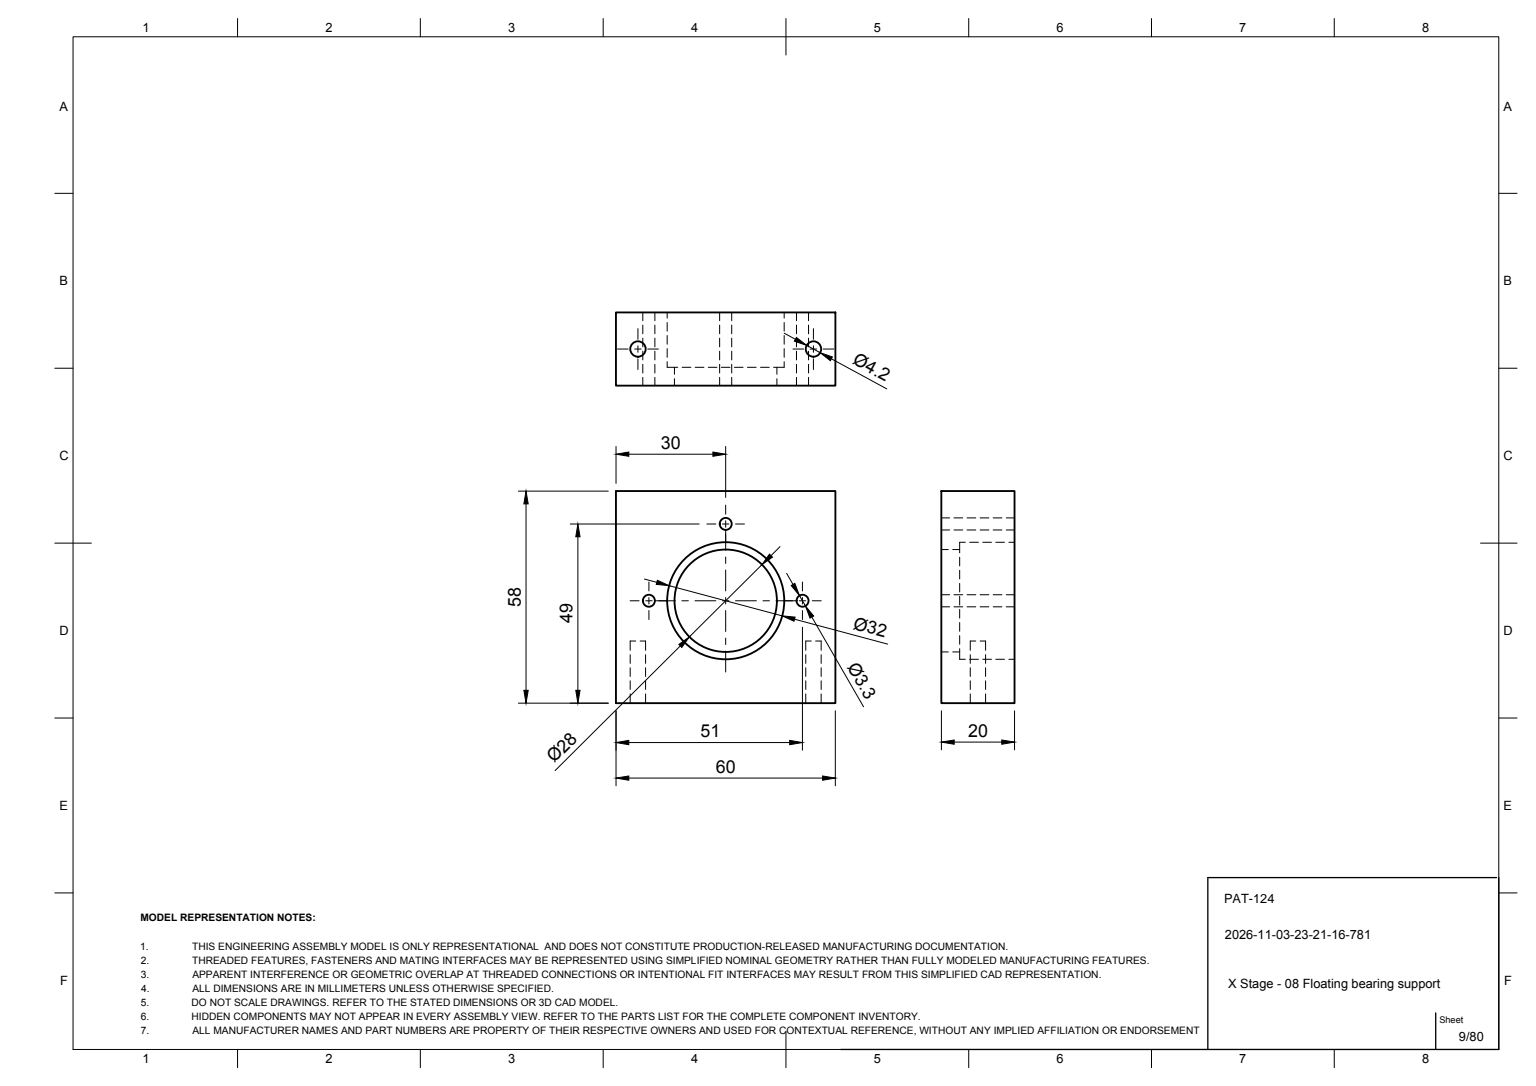
ISO-10303-21;
HEADER;
/* Generated by software containing ST-Developer
 * from STEP Tools, Inc. (www.steptools.com) 
 */

FILE_DESCRIPTION(
/* description */ ('XY cross-slide table'),
/* implementation_level */ '2;1');

FILE_NAME(
/* name */ 'X Stage - 08 Floating bearing support.step',
/* time_stamp */ '2026-10-28T03:22:46-07:00',
/* author */ (''),
/* organization */ (''),
/* preprocessor_version */ 'ST-DEVELOPER v20.2',
/* originating_system */ 'Autodesk Translation Framework v15.17.0.0',
/* authorisation */ '');

FILE_SCHEMA (('AUTOMOTIVE_DESIGN { 1 0 10303 214 3 1 1 }'));
ENDSEC;

DATA;
#10=MECHANICAL_DESIGN_GEOMETRIC_PRESENTATION_REPRESENTATION('',(#1674),#62984);
#1508=SHAPE_REPRESENTATION_RELATIONSHIP('SRR','None',#63356,#1591);
#1591=ADVANCED_BREP_SHAPE_REPRESENTATION('',(#1787),#62893);
#1674=STYLED_ITEM('',(#63912),#1787);
#1787=MANIFOLD_SOLID_BREP('Body1',#22968);
#1925=FACE_BOUND('',#4278,.T.);
#1926=FACE_BOUND('',#4286,.T.);
#1927=FACE_BOUND('',#4287,.T.);
#1928=FACE_BOUND('',#4288,.T.);
#1929=FACE_BOUND('',#4289,.T.);
#1930=FACE_BOUND('',#4292,.T.);
#1931=FACE_BOUND('',#4293,.T.);
#1932=FACE_BOUND('',#4294,.T.);
#1933=FACE_BOUND('',#4295,.T.);
#1934=FACE_BOUND('',#4298,.T.);
#1935=FACE_BOUND('',#4299,.T.);
#2324=PLANE('',#24120);
#2325=PLANE('',#24127);
#2326=PLANE('',#24131);
#2327=PLANE('',#24132);
#2328=PLANE('',#24133);
#2329=PLANE('',#24134);
#2330=PLANE('',#24135);
#2331=PLANE('',#24136);
#2332=PLANE('',#24137);
#2921=FACE_OUTER_BOUND('',#4273,.T.);
#2922=FACE_OUTER_BOUND('',#4274,.T.);
#2923=FACE_OUTER_BOUND('',#4275,.T.);
#2924=FACE_OUTER_BOUND('',#4276,.T.);
#2925=FACE_OUTER_BOUND('',#4277,.T.);
#2926=FACE_OUTER_BOUND('',#4279,.T.);
#2927=FACE_OUTER_BOUND('',#4280,.T.);
#2928=FACE_OUTER_BOUND('',#4281,.T.);
#2929=FACE_OUTER_BOUND('',#4282,.T.);
#2930=FACE_OUTER_BOUND('',#4283,.T.);
#2931=FACE_OUTER_BOUND('',#4284,.T.);
#2932=FACE_OUTER_BOUND('',#4285,.T.);
#2933=FACE_OUTER_BOUND('',#4290,.T.);
#2934=FACE_OUTER_BOUND('',#4291,.T.);
#2935=FACE_OUTER_BOUND('',#4296,.T.);
#2936=FACE_OUTER_BOUND('',#4297,.T.);
#4273=EDGE_LOOP('',(#15152,#15153,#15154,#15155));
#4274=EDGE_LOOP('',(#15156,#15157,#15158,#15159));
#4275=EDGE_LOOP('',(#15160,#15161,#15162,#15163));
#4276=EDGE_LOOP('',(#15164,#15165,#15166,#15167));
#4277=EDGE_LOOP('',(#15168));
#4278=EDGE_LOOP('',(#15169));
#4279=EDGE_LOOP('',(#15170,#15171,#15172,#15173));
#4280=EDGE_LOOP('',(#15174,#15175,#15176,#15177));
#4281=EDGE_LOOP('',(#15178));
#4282=EDGE_LOOP('',(#15179,#15180,#15181,#15182));
#4283=EDGE_LOOP('',(#15183));
#4284=EDGE_LOOP('',(#15184,#15185,#15186,#15187));
#4285=EDGE_LOOP('',(#15188,#15189,#15190,#15191));
#4286=EDGE_LOOP('',(#15192));
#4287=EDGE_LOOP('',(#15193));
#4288=EDGE_LOOP('',(#15194));
#4289=EDGE_LOOP('',(#15195));
#4290=EDGE_LOOP('',(#15196,#15197,#15198,#15199));
#4291=EDGE_LOOP('',(#15200,#15201,#15202,#15203));
#4292=EDGE_LOOP('',(#15204));
#4293=EDGE_LOOP('',(#15205));
#4294=EDGE_LOOP('',(#15206));
#4295=EDGE_LOOP('',(#15207));
#4296=EDGE_LOOP('',(#15208,#15209,#15210,#15211));
#4297=EDGE_LOOP('',(#15212,#15213,#15214,#15215));
#4298=EDGE_LOOP('',(#15216));
#4299=EDGE_LOOP('',(#15217));
#5982=LINE('',#33138,#7469);
#5983=LINE('',#33144,#7470);
#5984=LINE('',#33150,#7471);
#5985=LINE('',#33156,#7472);
#5986=LINE('',#33163,#7473);
#5987=LINE('',#33169,#7474);
#5988=LINE('',#33176,#7475);
#5989=LINE('',#33182,#7476);
#5990=LINE('',#33184,#7477);
#5991=LINE('',#33186,#7478);
#5992=LINE('',#33187,#7479);
#5993=LINE('',#33190,#7480);
#5994=LINE('',#33192,#7481);
#5995=LINE('',#33193,#7482);
#5996=LINE('',#33196,#7483);
#5997=LINE('',#33198,#7484);
#5998=LINE('',#33199,#7485);
#5999=LINE('',#33201,#7486);
#6000=LINE('',#33202,#7487);
#7469=VECTOR('',#26757,0.165);
#7470=VECTOR('',#26764,0.165);
#7471=VECTOR('',#26771,0.165);
#7472=VECTOR('',#26778,1.6);
#7473=VECTOR('',#26787,1.4);
#7474=VECTOR('',#26794,0.21);
#7475=VECTOR('',#26803,0.21);
#7476=VECTOR('',#26810,1.);
#7477=VECTOR('',#26811,1.);
#7478=VECTOR('',#26812,1.);
#7479=VECTOR('',#26813,1.);
#7480=VECTOR('',#26816,1.);
#7481=VECTOR('',#26817,1.);
#7482=VECTOR('',#26818,1.);
#7483=VECTOR('',#26821,1.);
#7484=VECTOR('',#26822,1.);
#7485=VECTOR('',#26823,1.);
#7486=VECTOR('',#26826,1.);
#7487=VECTOR('',#26827,1.);
#8928=CIRCLE('',#24109,0.165);
#8929=CIRCLE('',#24110,0.165);
#8930=CIRCLE('',#24112,0.165);
#8931=CIRCLE('',#24113,0.165);
#8932=CIRCLE('',#24115,0.165);
#8933=CIRCLE('',#24116,0.165);
#8934=CIRCLE('',#24118,1.6);
#8935=CIRCLE('',#24119,1.6);
#8936=CIRCLE('',#24121,1.4);
#8937=CIRCLE('',#24123,1.4);
#8938=CIRCLE('',#24125,0.21);
#8939=CIRCLE('',#24126,0.21);
#8940=CIRCLE('',#24129,0.21);
#8941=CIRCLE('',#24130,0.21);
#9853=VERTEX_POINT('',#33135);
#9854=VERTEX_POINT('',#33137);
#9855=VERTEX_POINT('',#33141);
#9856=VERTEX_POINT('',#33143);
#9857=VERTEX_POINT('',#33147);
#9858=VERTEX_POINT('',#33149);
#9859=VERTEX_POINT('',#33153);
#9860=VERTEX_POINT('',#33155);
#9861=VERTEX_POINT('',#33159);
#9862=VERTEX_POINT('',#33162);
#9863=VERTEX_POINT('',#33166);
#9864=VERTEX_POINT('',#33168);
#9865=VERTEX_POINT('',#33173);
#9866=VERTEX_POINT('',#33175);
#9867=VERTEX_POINT('',#33180);
#9868=VERTEX_POINT('',#33181);
#9869=VERTEX_POINT('',#33183);
#9870=VERTEX_POINT('',#33185);
#9871=VERTEX_POINT('',#33189);
#9872=VERTEX_POINT('',#33191);
#9873=VERTEX_POINT('',#33195);
#9874=VERTEX_POINT('',#33197);
#11960=EDGE_CURVE('',#9853,#9853,#8928,.T.);
#11961=EDGE_CURVE('',#9853,#9854,#5982,.T.);
#11962=EDGE_CURVE('',#9854,#9854,#8929,.T.);
#11963=EDGE_CURVE('',#9855,#9855,#8930,.T.);
#11964=EDGE_CURVE('',#9855,#9856,#5983,.T.);
#11965=EDGE_CURVE('',#9856,#9856,#8931,.T.);
#11966=EDGE_CURVE('',#9857,#9857,#8932,.T.);
#11967=EDGE_CURVE('',#9857,#9858,#5984,.T.);
#11968=EDGE_CURVE('',#9858,#9858,#8933,.T.);
#11969=EDGE_CURVE('',#9859,#9859,#8934,.T.);
#11970=EDGE_CURVE('',#9859,#9860,#5985,.T.);
#11971=EDGE_CURVE('',#9860,#9860,#8935,.T.);
#11972=EDGE_CURVE('',#9861,#9861,#8936,.T.);
#11973=EDGE_CURVE('',#9861,#9862,#5986,.T.);
#11974=EDGE_CURVE('',#9862,#9862,#8937,.T.);
#11975=EDGE_CURVE('',#9863,#9863,#8938,.T.);
#11976=EDGE_CURVE('',#9863,#9864,#5987,.T.);
#11977=EDGE_CURVE('',#9864,#9864,#8939,.T.);
#11978=EDGE_CURVE('',#9865,#9865,#8940,.T.);
#11979=EDGE_CURVE('',#9865,#9866,#5988,.T.);
#11980=EDGE_CURVE('',#9866,#9866,#8941,.T.);
#11981=EDGE_CURVE('',#9867,#9868,#5989,.T.);
#11982=EDGE_CURVE('',#9868,#9869,#5990,.T.);
#11983=EDGE_CURVE('',#9870,#9869,#5991,.T.);
#11984=EDGE_CURVE('',#9867,#9870,#5992,.T.);
#11985=EDGE_CURVE('',#9871,#9867,#5993,.T.);
#11986=EDGE_CURVE('',#9872,#9870,#5994,.T.);
#11987=EDGE_CURVE('',#9871,#9872,#5995,.T.);
#11988=EDGE_CURVE('',#9873,#9871,#5996,.T.);
#11989=EDGE_CURVE('',#9874,#9872,#5997,.T.);
#11990=EDGE_CURVE('',#9873,#9874,#5998,.T.);
#11991=EDGE_CURVE('',#9868,#9873,#5999,.T.);
#11992=EDGE_CURVE('',#9869,#9874,#6000,.T.);
#15152=ORIENTED_EDGE('',*,*,#11960,.F.);
#15153=ORIENTED_EDGE('',*,*,#11961,.T.);
#15154=ORIENTED_EDGE('',*,*,#11962,.F.);
#15155=ORIENTED_EDGE('',*,*,#11961,.F.);
#15156=ORIENTED_EDGE('',*,*,#11963,.F.);
#15157=ORIENTED_EDGE('',*,*,#11964,.T.);
#15158=ORIENTED_EDGE('',*,*,#11965,.F.);
#15159=ORIENTED_EDGE('',*,*,#11964,.F.);
#15160=ORIENTED_EDGE('',*,*,#11966,.F.);
#15161=ORIENTED_EDGE('',*,*,#11967,.T.);
#15162=ORIENTED_EDGE('',*,*,#11968,.F.);
#15163=ORIENTED_EDGE('',*,*,#11967,.F.);
#15164=ORIENTED_EDGE('',*,*,#11969,.F.);
#15165=ORIENTED_EDGE('',*,*,#11970,.T.);
#15166=ORIENTED_EDGE('',*,*,#11971,.T.);
#15167=ORIENTED_EDGE('',*,*,#11970,.F.);
#15168=ORIENTED_EDGE('',*,*,#11971,.F.);
#15169=ORIENTED_EDGE('',*,*,#11972,.F.);
#15170=ORIENTED_EDGE('',*,*,#11972,.T.);
#15171=ORIENTED_EDGE('',*,*,#11973,.T.);
#15172=ORIENTED_EDGE('',*,*,#11974,.F.);
#15173=ORIENTED_EDGE('',*,*,#11973,.F.);
#15174=ORIENTED_EDGE('',*,*,#11975,.F.);
#15175=ORIENTED_EDGE('',*,*,#11976,.T.);
#15176=ORIENTED_EDGE('',*,*,#11977,.T.);
#15177=ORIENTED_EDGE('',*,*,#11976,.F.);
#15178=ORIENTED_EDGE('',*,*,#11977,.F.);
#15179=ORIENTED_EDGE('',*,*,#11978,.F.);
#15180=ORIENTED_EDGE('',*,*,#11979,.T.);
#15181=ORIENTED_EDGE('',*,*,#11980,.T.);
#15182=ORIENTED_EDGE('',*,*,#11979,.F.);
#15183=ORIENTED_EDGE('',*,*,#11980,.F.);
#15184=ORIENTED_EDGE('',*,*,#11981,.T.);
#15185=ORIENTED_EDGE('',*,*,#11982,.T.);
#15186=ORIENTED_EDGE('',*,*,#11983,.F.);
#15187=ORIENTED_EDGE('',*,*,#11984,.F.);
#15188=ORIENTED_EDGE('',*,*,#11985,.T.);
#15189=ORIENTED_EDGE('',*,*,#11984,.T.);
#15190=ORIENTED_EDGE('',*,*,#11986,.F.);
#15191=ORIENTED_EDGE('',*,*,#11987,.F.);
#15192=ORIENTED_EDGE('',*,*,#11962,.T.);
#15193=ORIENTED_EDGE('',*,*,#11965,.T.);
#15194=ORIENTED_EDGE('',*,*,#11968,.T.);
#15195=ORIENTED_EDGE('',*,*,#11974,.T.);
#15196=ORIENTED_EDGE('',*,*,#11988,.T.);
#15197=ORIENTED_EDGE('',*,*,#11987,.T.);
#15198=ORIENTED_EDGE('',*,*,#11989,.F.);
#15199=ORIENTED_EDGE('',*,*,#11990,.F.);
#15200=ORIENTED_EDGE('',*,*,#11991,.T.);
#15201=ORIENTED_EDGE('',*,*,#11990,.T.);
#15202=ORIENTED_EDGE('',*,*,#11992,.F.);
#15203=ORIENTED_EDGE('',*,*,#11982,.F.);
#15204=ORIENTED_EDGE('',*,*,#11960,.T.);
#15205=ORIENTED_EDGE('',*,*,#11963,.T.);
#15206=ORIENTED_EDGE('',*,*,#11966,.T.);
#15207=ORIENTED_EDGE('',*,*,#11969,.T.);
#15208=ORIENTED_EDGE('',*,*,#11992,.T.);
#15209=ORIENTED_EDGE('',*,*,#11989,.T.);
#15210=ORIENTED_EDGE('',*,*,#11986,.T.);
#15211=ORIENTED_EDGE('',*,*,#11983,.T.);
#15212=ORIENTED_EDGE('',*,*,#11991,.F.);
#15213=ORIENTED_EDGE('',*,*,#11981,.F.);
#15214=ORIENTED_EDGE('',*,*,#11985,.F.);
#15215=ORIENTED_EDGE('',*,*,#11988,.F.);
#15216=ORIENTED_EDGE('',*,*,#11975,.T.);
#15217=ORIENTED_EDGE('',*,*,#11978,.T.);
#21064=CYLINDRICAL_SURFACE('',#24108,0.165);
#21065=CYLINDRICAL_SURFACE('',#24111,0.165);
#21066=CYLINDRICAL_SURFACE('',#24114,0.165);
#21067=CYLINDRICAL_SURFACE('',#24117,1.6);
#21068=CYLINDRICAL_SURFACE('',#24122,1.4);
#21069=CYLINDRICAL_SURFACE('',#24124,0.21);
#21070=CYLINDRICAL_SURFACE('',#24128,0.21);
#21702=ADVANCED_FACE('',(#2921),#21064,.F.);
#21703=ADVANCED_FACE('',(#2922),#21065,.F.);
#21704=ADVANCED_FACE('',(#2923),#21066,.F.);
#21705=ADVANCED_FACE('',(#2924),#21067,.F.);
#21706=ADVANCED_FACE('',(#2925,#1925),#2324,.F.);
#21707=ADVANCED_FACE('',(#2926),#21068,.F.);
#21708=ADVANCED_FACE('',(#2927),#21069,.F.);
#21709=ADVANCED_FACE('',(#2928),#2325,.F.);
#21710=ADVANCED_FACE('',(#2929),#21070,.F.);
#21711=ADVANCED_FACE('',(#2930),#2326,.F.);
#21712=ADVANCED_FACE('',(#2931),#2327,.T.);
#21713=ADVANCED_FACE('',(#2932,#1926,#1927,#1928,#1929),#2328,.T.);
#21714=ADVANCED_FACE('',(#2933),#2329,.T.);
#21715=ADVANCED_FACE('',(#2934,#1930,#1931,#1932,#1933),#2330,.T.);
#21716=ADVANCED_FACE('',(#2935),#2331,.T.);
#21717=ADVANCED_FACE('',(#2936,#1934,#1935),#2332,.F.);
#22968=CLOSED_SHELL('',(#21702,#21703,#21704,#21705,#21706,#21707,#21708,
#21709,#21710,#21711,#21712,#21713,#21714,#21715,#21716,#21717));
#24107=AXIS2_PLACEMENT_3D('',#33133,#26751,#26752);
#24108=AXIS2_PLACEMENT_3D('',#33134,#26753,#26754);
#24109=AXIS2_PLACEMENT_3D('',#33136,#26755,#26756);
#24110=AXIS2_PLACEMENT_3D('',#33139,#26758,#26759);
#24111=AXIS2_PLACEMENT_3D('',#33140,#26760,#26761);
#24112=AXIS2_PLACEMENT_3D('',#33142,#26762,#26763);
#24113=AXIS2_PLACEMENT_3D('',#33145,#26765,#26766);
#24114=AXIS2_PLACEMENT_3D('',#33146,#26767,#26768);
#24115=AXIS2_PLACEMENT_3D('',#33148,#26769,#26770);
#24116=AXIS2_PLACEMENT_3D('',#33151,#26772,#26773);
#24117=AXIS2_PLACEMENT_3D('',#33152,#26774,#26775);
#24118=AXIS2_PLACEMENT_3D('',#33154,#26776,#26777);
#24119=AXIS2_PLACEMENT_3D('',#33157,#26779,#26780);
#24120=AXIS2_PLACEMENT_3D('',#33158,#26781,#26782);
#24121=AXIS2_PLACEMENT_3D('',#33160,#26783,#26784);
#24122=AXIS2_PLACEMENT_3D('',#33161,#26785,#26786);
#24123=AXIS2_PLACEMENT_3D('',#33164,#26788,#26789);
#24124=AXIS2_PLACEMENT_3D('',#33165,#26790,#26791);
#24125=AXIS2_PLACEMENT_3D('',#33167,#26792,#26793);
#24126=AXIS2_PLACEMENT_3D('',#33170,#26795,#26796);
#24127=AXIS2_PLACEMENT_3D('',#33171,#26797,#26798);
#24128=AXIS2_PLACEMENT_3D('',#33172,#26799,#26800);
#24129=AXIS2_PLACEMENT_3D('',#33174,#26801,#26802);
#24130=AXIS2_PLACEMENT_3D('',#33177,#26804,#26805);
#24131=AXIS2_PLACEMENT_3D('',#33178,#26806,#26807);
#24132=AXIS2_PLACEMENT_3D('',#33179,#26808,#26809);
#24133=AXIS2_PLACEMENT_3D('',#33188,#26814,#26815);
#24134=AXIS2_PLACEMENT_3D('',#33194,#26819,#26820);
#24135=AXIS2_PLACEMENT_3D('',#33200,#26824,#26825);
#24136=AXIS2_PLACEMENT_3D('',#33203,#26828,#26829);
#24137=AXIS2_PLACEMENT_3D('',#33204,#26830,#26831);
#26751=DIRECTION('axis',(0.,0.,1.));
#26752=DIRECTION('refdir',(1.,0.,0.));
#26753=DIRECTION('center_axis',(1.,0.,0.));
#26754=DIRECTION('ref_axis',(0.,0.,-1.));
#26755=DIRECTION('center_axis',(1.,0.,0.));
#26756=DIRECTION('ref_axis',(0.,0.,-1.));
#26757=DIRECTION('',(1.,0.,0.));
#26758=DIRECTION('center_axis',(-1.,0.,0.));
#26759=DIRECTION('ref_axis',(0.,0.,-1.));
#26760=DIRECTION('center_axis',(1.,0.,0.));
#26761=DIRECTION('ref_axis',(0.,0.,-1.));
#26762=DIRECTION('center_axis',(1.,0.,0.));
#26763=DIRECTION('ref_axis',(0.,0.,-1.));
#26764=DIRECTION('',(1.,0.,0.));
#26765=DIRECTION('center_axis',(-1.,0.,0.));
#26766=DIRECTION('ref_axis',(0.,0.,-1.));
#26767=DIRECTION('center_axis',(1.,0.,0.));
#26768=DIRECTION('ref_axis',(0.,0.,-1.));
#26769=DIRECTION('center_axis',(1.,0.,0.));
#26770=DIRECTION('ref_axis',(0.,0.,-1.));
#26771=DIRECTION('',(1.,0.,0.));
#26772=DIRECTION('center_axis',(-1.,0.,0.));
#26773=DIRECTION('ref_axis',(0.,0.,-1.));
#26774=DIRECTION('center_axis',(1.,0.,0.));
#26775=DIRECTION('ref_axis',(0.,0.,-1.));
#26776=DIRECTION('center_axis',(1.,0.,0.));
#26777=DIRECTION('ref_axis',(0.,0.,-1.));
#26778=DIRECTION('',(1.,0.,0.));
#26779=DIRECTION('center_axis',(1.,0.,0.));
#26780=DIRECTION('ref_axis',(0.,0.,-1.));
#26781=DIRECTION('center_axis',(1.,0.,0.));
#26782=DIRECTION('ref_axis',(0.,0.,-1.));
#26783=DIRECTION('center_axis',(-1.,0.,0.));
#26784=DIRECTION('ref_axis',(0.,0.,-1.));
#26785=DIRECTION('center_axis',(1.,0.,0.));
#26786=DIRECTION('ref_axis',(0.,0.,-1.));
#26787=DIRECTION('',(1.,0.,0.));
#26788=DIRECTION('center_axis',(-1.,0.,0.));
#26789=DIRECTION('ref_axis',(0.,0.,-1.));
#26790=DIRECTION('center_axis',(0.,0.,1.));
#26791=DIRECTION('ref_axis',(1.,0.,0.));
#26792=DIRECTION('center_axis',(0.,0.,1.));
#26793=DIRECTION('ref_axis',(1.,0.,0.));
#26794=DIRECTION('',(0.,0.,1.));
#26795=DIRECTION('center_axis',(0.,0.,1.));
#26796=DIRECTION('ref_axis',(1.,0.,0.));
#26797=DIRECTION('center_axis',(0.,0.,1.));
#26798=DIRECTION('ref_axis',(1.,0.,0.));
#26799=DIRECTION('center_axis',(0.,0.,1.));
#26800=DIRECTION('ref_axis',(1.,0.,0.));
#26801=DIRECTION('center_axis',(0.,0.,1.));
#26802=DIRECTION('ref_axis',(1.,0.,0.));
#26803=DIRECTION('',(0.,0.,1.));
#26804=DIRECTION('center_axis',(0.,0.,1.));
#26805=DIRECTION('ref_axis',(1.,0.,0.));
#26806=DIRECTION('center_axis',(0.,0.,1.));
#26807=DIRECTION('ref_axis',(1.,0.,0.));
#26808=DIRECTION('center_axis',(0.,1.,0.));
#26809=DIRECTION('ref_axis',(-1.,0.,0.));
#26810=DIRECTION('',(-1.,0.,0.));
#26811=DIRECTION('',(0.,0.,1.));
#26812=DIRECTION('',(-1.,0.,0.));
#26813=DIRECTION('',(0.,0.,1.));
#26814=DIRECTION('center_axis',(1.,0.,0.));
#26815=DIRECTION('ref_axis',(0.,1.,0.));
#26816=DIRECTION('',(0.,1.,0.));
#26817=DIRECTION('',(0.,1.,0.));
#26818=DIRECTION('',(0.,0.,1.));
#26819=DIRECTION('center_axis',(0.,-1.,0.));
#26820=DIRECTION('ref_axis',(1.,0.,0.));
#26821=DIRECTION('',(1.,0.,0.));
#26822=DIRECTION('',(1.,0.,0.));
#26823=DIRECTION('',(0.,0.,1.));
#26824=DIRECTION('center_axis',(-1.,0.,0.));
#26825=DIRECTION('ref_axis',(0.,-1.,0.));
#26826=DIRECTION('',(0.,-1.,0.));
#26827=DIRECTION('',(0.,-1.,0.));
#26828=DIRECTION('center_axis',(0.,0.,1.));
#26829=DIRECTION('ref_axis',(1.,0.,0.));
#26830=DIRECTION('center_axis',(0.,0.,1.));
#26831=DIRECTION('ref_axis',(1.,0.,0.));
#33133=CARTESIAN_POINT('',(0.,0.,0.));
#33134=CARTESIAN_POINT('Origin',(1.9,-2.1,4.));
#33135=CARTESIAN_POINT('',(2.,-2.1,4.165));
#33136=CARTESIAN_POINT('Origin',(2.,-2.1,4.));
#33137=CARTESIAN_POINT('',(4.,-2.1,4.165));
#33138=CARTESIAN_POINT('',(1.9,-2.1,4.165));
#33139=CARTESIAN_POINT('Origin',(4.,-2.1,4.));
#33140=CARTESIAN_POINT('Origin',(1.9,2.1,4.));
#33141=CARTESIAN_POINT('',(2.,2.1,4.165));
#33142=CARTESIAN_POINT('Origin',(2.,2.1,4.));
#33143=CARTESIAN_POINT('',(4.,2.1,4.165));
#33144=CARTESIAN_POINT('',(1.9,2.1,4.165));
#33145=CARTESIAN_POINT('Origin',(4.,2.1,4.));
#33146=CARTESIAN_POINT('Origin',(1.9,0.,6.1));
#33147=CARTESIAN_POINT('',(2.,-2.02066721859313E-17,6.265));
#33148=CARTESIAN_POINT('Origin',(2.,0.,6.1));
#33149=CARTESIAN_POINT('',(4.,2.02066721859313E-17,6.265));
#33150=CARTESIAN_POINT('',(1.9,-2.02066721859313E-17,6.265));
#33151=CARTESIAN_POINT('Origin',(4.,0.,6.1));
#33152=CARTESIAN_POINT('Origin',(1.9,0.,4.));
#33153=CARTESIAN_POINT('',(2.,-1.95943487863577E-16,5.6));
#33154=CARTESIAN_POINT('Origin',(2.,0.,4.));
#33155=CARTESIAN_POINT('',(3.5,-1.95943487863577E-16,5.6));
#33156=CARTESIAN_POINT('',(1.9,-1.95943487863577E-16,5.6));
#33157=CARTESIAN_POINT('Origin',(3.5,0.,4.));
#33158=CARTESIAN_POINT('Origin',(3.5,0.,4.));
#33159=CARTESIAN_POINT('',(3.5,1.71450551880629E-16,5.4));
#33160=CARTESIAN_POINT('Origin',(3.5,0.,4.));
#33161=CARTESIAN_POINT('Origin',(1.9,0.,4.));
#33162=CARTESIAN_POINT('',(4.,1.71450551880629E-16,5.4));
#33163=CARTESIAN_POINT('',(1.9,-1.71450551880629E-16,5.4));
#33164=CARTESIAN_POINT('Origin',(4.,0.,4.));
#33165=CARTESIAN_POINT('Origin',(3.,-2.4,1.1));
#33166=CARTESIAN_POINT('',(2.79,-2.4,1.2));
#33167=CARTESIAN_POINT('Origin',(3.,-2.4,1.2));
#33168=CARTESIAN_POINT('',(2.79,-2.4,2.9));
#33169=CARTESIAN_POINT('',(2.79,-2.4,1.1));
#33170=CARTESIAN_POINT('Origin',(3.,-2.4,2.9));
#33171=CARTESIAN_POINT('Origin',(3.,-2.4,2.9));
#33172=CARTESIAN_POINT('Origin',(3.,2.4,1.1));
#33173=CARTESIAN_POINT('',(2.79,2.4,1.2));
#33174=CARTESIAN_POINT('Origin',(3.,2.4,1.2));
#33175=CARTESIAN_POINT('',(2.79,2.4,2.9));
#33176=CARTESIAN_POINT('',(2.79,2.4,1.1));
#33177=CARTESIAN_POINT('Origin',(3.,2.4,2.9));
#33178=CARTESIAN_POINT('Origin',(3.,2.4,2.9));
#33179=CARTESIAN_POINT('Origin',(4.,3.,1.2));
#33180=CARTESIAN_POINT('',(4.,3.,1.2));
#33181=CARTESIAN_POINT('',(2.,3.,1.2));
#33182=CARTESIAN_POINT('',(4.,3.,1.2));
#33183=CARTESIAN_POINT('',(2.,3.,7.));
#33184=CARTESIAN_POINT('',(2.,3.,1.2));
#33185=CARTESIAN_POINT('',(4.,3.,7.));
#33186=CARTESIAN_POINT('',(4.,3.,7.));
#33187=CARTESIAN_POINT('',(4.,3.,1.2));
#33188=CARTESIAN_POINT('Origin',(4.,-3.,1.2));
#33189=CARTESIAN_POINT('',(4.,-3.,1.2));
#33190=CARTESIAN_POINT('',(4.,-3.,1.2));
#33191=CARTESIAN_POINT('',(4.,-3.,7.));
#33192=CARTESIAN_POINT('',(4.,-3.,7.));
#33193=CARTESIAN_POINT('',(4.,-3.,1.2));
#33194=CARTESIAN_POINT('Origin',(2.,-3.,1.2));
#33195=CARTESIAN_POINT('',(2.,-3.,1.2));
#33196=CARTESIAN_POINT('',(2.,-3.,1.2));
#33197=CARTESIAN_POINT('',(2.,-3.,7.));
#33198=CARTESIAN_POINT('',(2.,-3.,7.));
#33199=CARTESIAN_POINT('',(2.,-3.,1.2));
#33200=CARTESIAN_POINT('Origin',(2.,3.,1.2));
#33201=CARTESIAN_POINT('',(2.,3.,1.2));
#33202=CARTESIAN_POINT('',(2.,3.,7.));
#33203=CARTESIAN_POINT('Origin',(3.,0.,7.));
#33204=CARTESIAN_POINT('Origin',(3.,0.,1.2));
#62794=UNCERTAINTY_MEASURE_WITH_UNIT(LENGTH_MEASURE(0.001),#62985,
'DISTANCE_ACCURACY_VALUE',
'Maximum model space distance between geometric entities at asserted c
onnectivities');
#62885=UNCERTAINTY_MEASURE_WITH_UNIT(LENGTH_MEASURE(0.001),#62985,
'DISTANCE_ACCURACY_VALUE',
'Maximum model space distance between geometric entities at asserted c
onnectivities');
#62893=(
GEOMETRIC_REPRESENTATION_CONTEXT(3)
GLOBAL_UNCERTAINTY_ASSIGNED_CONTEXT((#62794))
GLOBAL_UNIT_ASSIGNED_CONTEXT((#62985,#62987,#62988))
REPRESENTATION_CONTEXT('','3D')
);
#62984=(
GEOMETRIC_REPRESENTATION_CONTEXT(3)
GLOBAL_UNCERTAINTY_ASSIGNED_CONTEXT((#62885))
GLOBAL_UNIT_ASSIGNED_CONTEXT((#62985,#62987,#62988))
REPRESENTATION_CONTEXT('','3D')
);
#62985=(
LENGTH_UNIT()
NAMED_UNIT(*)
SI_UNIT(.CENTI.,.METRE.)
);
#62987=(
NAMED_UNIT(*)
PLANE_ANGLE_UNIT()
SI_UNIT($,.RADIAN.)
);
#62988=(
NAMED_UNIT(*)
SI_UNIT($,.STERADIAN.)
SOLID_ANGLE_UNIT()
);
#62996=SHAPE_DEFINITION_REPRESENTATION(#63094,#63356);
#63094=PRODUCT_DEFINITION_SHAPE('',$,#63455);
#63356=SHAPE_REPRESENTATION('',(#24107),#62893);
#63447=PRODUCT_DEFINITION_CONTEXT('part definition',#63743,'design');
#63455=PRODUCT_DEFINITION('X Stage - 08 Floating bearing support',
'X Stage - 08 Floating bearing support',#63553,#63447);
#63553=PRODUCT_DEFINITION_FORMATION('',$,#63752);
#63743=APPLICATION_CONTEXT(
'Core Data for Automotive Mechanical Design Process');
#63744=PRODUCT_CONTEXT('part definition',#63743,'mechanical');
#63752=PRODUCT('X Stage - 08 Floating bearing support',
'X Stage - 08 Floating bearing support',
'X Stage - 08 Floating bearing support',(#63744));
#63906=COLOUR_RGB('Grey',0.48,0.52,0.57);
#63907=FILL_AREA_STYLE_COLOUR('',#63906);
#63908=FILL_AREA_STYLE('',(#63907));
#63909=SURFACE_STYLE_FILL_AREA(#63908);
#63910=SURFACE_SIDE_STYLE('',(#63909));
#63911=SURFACE_STYLE_USAGE(.BOTH.,#63910);
#63912=PRESENTATION_STYLE_ASSIGNMENT((#63911));
ENDSEC;
END-ISO-10303-21;
